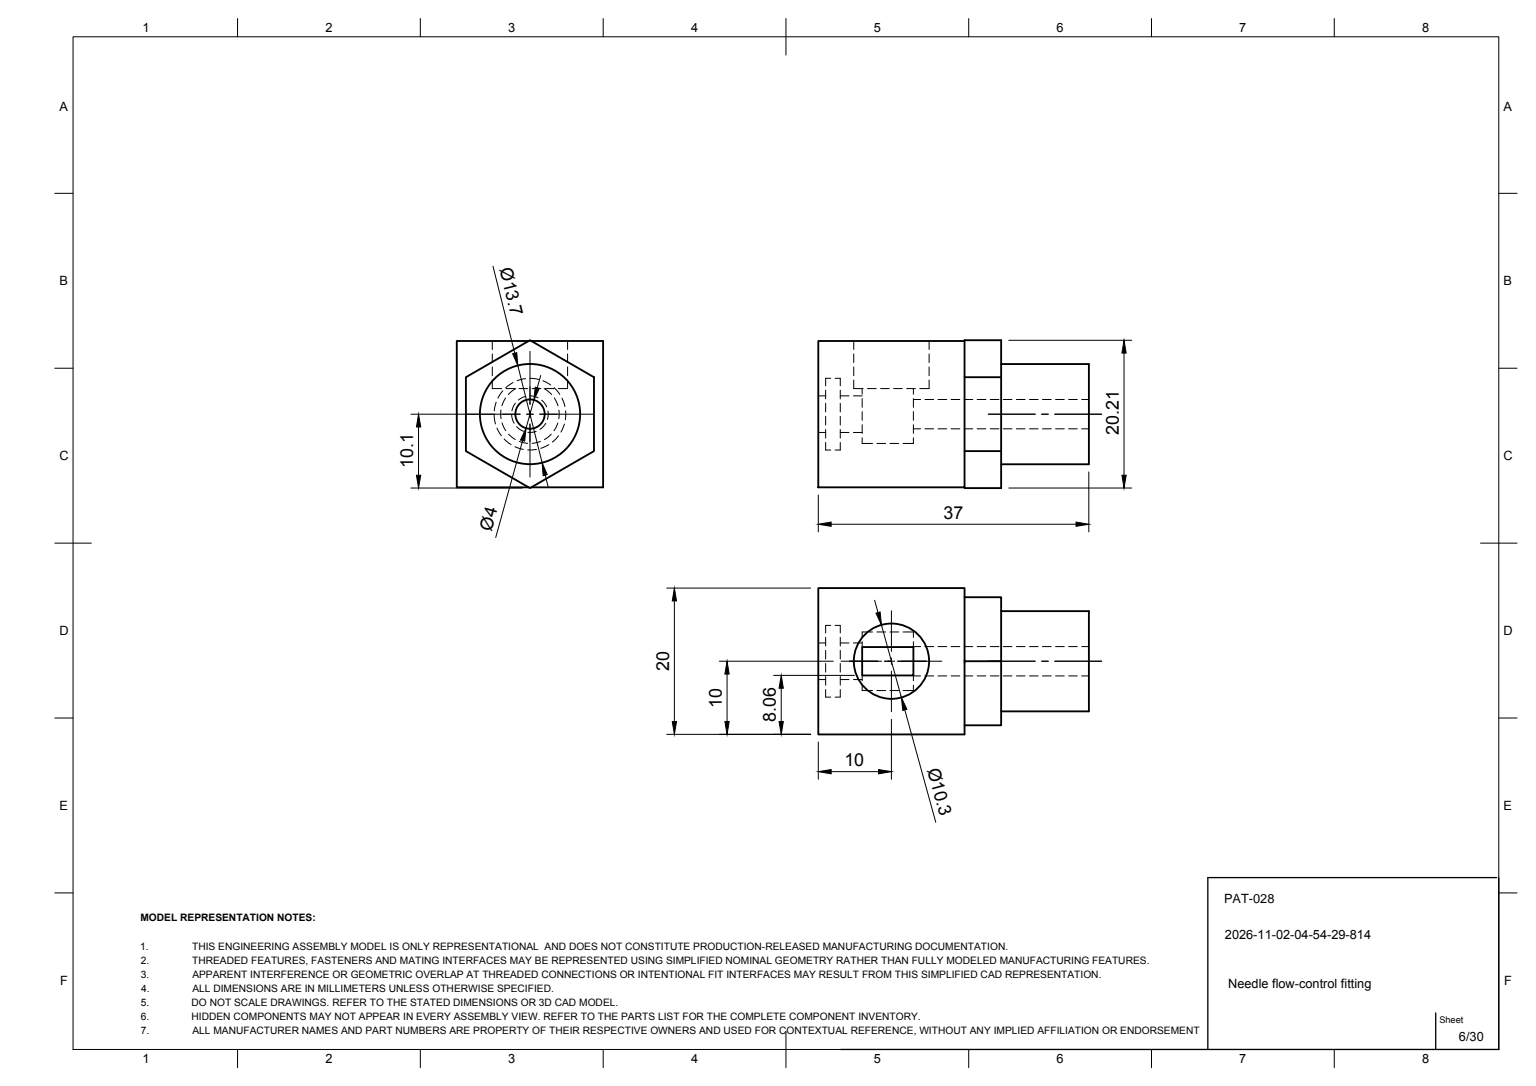
ISO-10303-21;
HEADER;
/* Generated by software containing ST-Developer
 * from STEP Tools, Inc. (www.steptools.com) 
 */

FILE_DESCRIPTION(
/* description */ ('Cylinder foot and clevis mount kit'),
/* implementation_level */ '2;1');

FILE_NAME(
/* name */ 'Needle flow-control fitting.step',
/* time_stamp */ '2026-10-27T20:10:43-07:00',
/* author */ (''),
/* organization */ (''),
/* preprocessor_version */ 'ST-DEVELOPER v20.2',
/* originating_system */ 'Autodesk Translation Framework v15.17.0.0',
/* authorisation */ '');

FILE_SCHEMA (('AUTOMOTIVE_DESIGN { 1 0 10303 214 3 1 1 }'));
ENDSEC;

DATA;
#10=MECHANICAL_DESIGN_GEOMETRIC_PRESENTATION_REPRESENTATION('',(#339),#9102);
#283=SHAPE_REPRESENTATION_RELATIONSHIP('SRR','None',#9230,#311);
#311=ADVANCED_BREP_SHAPE_REPRESENTATION('',(#367),#9073);
#339=STYLED_ITEM('',(#9453),#367);
#367=MANIFOLD_SOLID_BREP('Body1',#4925);
#407=FACE_BOUND('',#1050,.T.);
#408=FACE_BOUND('',#1052,.T.);
#409=FACE_BOUND('',#1056,.T.);
#410=FACE_BOUND('',#1058,.T.);
#411=FACE_BOUND('',#1062,.T.);
#412=FACE_BOUND('',#1066,.T.);
#413=FACE_BOUND('',#1070,.T.);
#414=FACE_BOUND('',#1074,.T.);
#415=FACE_BOUND('',#1085,.T.);
#526=PLANE('',#5339);
#527=PLANE('',#5340);
#528=PLANE('',#5348);
#529=PLANE('',#5350);
#530=PLANE('',#5355);
#531=PLANE('',#5357);
#532=PLANE('',#5358);
#533=PLANE('',#5359);
#534=PLANE('',#5360);
#535=PLANE('',#5361);
#536=PLANE('',#5362);
#537=PLANE('',#5363);
#538=PLANE('',#5364);
#539=PLANE('',#5365);
#540=PLANE('',#5367);
#541=PLANE('',#5368);
#542=PLANE('',#5369);
#543=PLANE('',#5370);
#544=PLANE('',#5371);
#545=PLANE('',#5372);
#546=PLANE('',#5373);
#547=PLANE('',#5378);
#727=FACE_OUTER_BOUND('',#1048,.T.);
#728=FACE_OUTER_BOUND('',#1049,.T.);
#729=FACE_OUTER_BOUND('',#1051,.T.);
#730=FACE_OUTER_BOUND('',#1053,.T.);
#731=FACE_OUTER_BOUND('',#1054,.T.);
#732=FACE_OUTER_BOUND('',#1055,.T.);
#733=FACE_OUTER_BOUND('',#1057,.T.);
#734=FACE_OUTER_BOUND('',#1059,.T.);
#735=FACE_OUTER_BOUND('',#1060,.T.);
#736=FACE_OUTER_BOUND('',#1061,.T.);
#737=FACE_OUTER_BOUND('',#1063,.T.);
#738=FACE_OUTER_BOUND('',#1064,.T.);
#739=FACE_OUTER_BOUND('',#1065,.T.);
#740=FACE_OUTER_BOUND('',#1067,.T.);
#741=FACE_OUTER_BOUND('',#1068,.T.);
#742=FACE_OUTER_BOUND('',#1069,.T.);
#743=FACE_OUTER_BOUND('',#1071,.T.);
#744=FACE_OUTER_BOUND('',#1072,.T.);
#745=FACE_OUTER_BOUND('',#1073,.T.);
#746=FACE_OUTER_BOUND('',#1075,.T.);
#747=FACE_OUTER_BOUND('',#1076,.T.);
#748=FACE_OUTER_BOUND('',#1077,.T.);
#749=FACE_OUTER_BOUND('',#1078,.T.);
#750=FACE_OUTER_BOUND('',#1079,.T.);
#751=FACE_OUTER_BOUND('',#1080,.T.);
#752=FACE_OUTER_BOUND('',#1081,.T.);
#753=FACE_OUTER_BOUND('',#1082,.T.);
#754=FACE_OUTER_BOUND('',#1083,.T.);
#755=FACE_OUTER_BOUND('',#1084,.T.);
#1048=EDGE_LOOP('',(#3449,#3450,#3451,#3452));
#1049=EDGE_LOOP('',(#3453));
#1050=EDGE_LOOP('',(#3454,#3455,#3456,#3457));
#1051=EDGE_LOOP('',(#3458,#3459));
#1052=EDGE_LOOP('',(#3460));
#1053=EDGE_LOOP('',(#3461,#3462,#3463,#3464));
#1054=EDGE_LOOP('',(#3465,#3466,#3467,#3468));
#1055=EDGE_LOOP('',(#3469));
#1056=EDGE_LOOP('',(#3470));
#1057=EDGE_LOOP('',(#3471));
#1058=EDGE_LOOP('',(#3472));
#1059=EDGE_LOOP('',(#3473,#3474,#3475,#3476));
#1060=EDGE_LOOP('',(#3477,#3478,#3479,#3480));
#1061=EDGE_LOOP('',(#3481,#3482));
#1062=EDGE_LOOP('',(#3483));
#1063=EDGE_LOOP('',(#3484,#3485,#3486,#3487,#3488,#3489));
#1064=EDGE_LOOP('',(#3490,#3491,#3492,#3493));
#1065=EDGE_LOOP('',(#3494,#3495,#3496,#3497,#3498,#3499));
#1066=EDGE_LOOP('',(#3500));
#1067=EDGE_LOOP('',(#3501,#3502,#3503,#3504));
#1068=EDGE_LOOP('',(#3505,#3506,#3507,#3508,#3509,#3510));
#1069=EDGE_LOOP('',(#3511,#3512,#3513,#3514));
#1070=EDGE_LOOP('',(#3515));
#1071=EDGE_LOOP('',(#3516,#3517,#3518,#3519,#3520,#3521));
#1072=EDGE_LOOP('',(#3522,#3523,#3524));
#1073=EDGE_LOOP('',(#3525,#3526,#3527,#3528,#3529,#3530));
#1074=EDGE_LOOP('',(#3531));
#1075=EDGE_LOOP('',(#3532,#3533,#3534,#3535));
#1076=EDGE_LOOP('',(#3536,#3537,#3538,#3539,#3540));
#1077=EDGE_LOOP('',(#3541,#3542,#3543,#3544,#3545));
#1078=EDGE_LOOP('',(#3546,#3547,#3548,#3549));
#1079=EDGE_LOOP('',(#3550,#3551,#3552,#3553,#3554));
#1080=EDGE_LOOP('',(#3555,#3556,#3557,#3558,#3559));
#1081=EDGE_LOOP('',(#3560,#3561,#3562));
#1082=EDGE_LOOP('',(#3563,#3564,#3565,#3566));
#1083=EDGE_LOOP('',(#3567,#3568,#3569,#3570));
#1084=EDGE_LOOP('',(#3571));
#1085=EDGE_LOOP('',(#3572));
#1440=LINE('',#7643,#1789);
#1441=LINE('',#7648,#1790);
#1442=LINE('',#7650,#1791);
#1443=LINE('',#7652,#1792);
#1444=LINE('',#7653,#1793);
#1445=LINE('',#7664,#1794);
#1446=LINE('',#7673,#1795);
#1447=LINE('',#7676,#1796);
#1448=LINE('',#7684,#1797);
#1449=LINE('',#7686,#1798);
#1450=LINE('',#7688,#1799);
#1451=LINE('',#7690,#1800);
#1452=LINE('',#7692,#1801);
#1453=LINE('',#7693,#1802);
#1454=LINE('',#7697,#1803);
#1455=LINE('',#7699,#1804);
#1456=LINE('',#7701,#1805);
#1457=LINE('',#7702,#1806);
#1458=LINE('',#7705,#1807);
#1459=LINE('',#7706,#1808);
#1460=LINE('',#7708,#1809);
#1461=LINE('',#7709,#1810);
#1462=LINE('',#7712,#1811);
#1463=LINE('',#7713,#1812);
#1464=LINE('',#7716,#1813);
#1465=LINE('',#7717,#1814);
#1466=LINE('',#7718,#1815);
#1467=LINE('',#7722,#1816);
#1468=LINE('',#7724,#1817);
#1469=LINE('',#7725,#1818);
#1470=LINE('',#7728,#1819);
#1471=LINE('',#7729,#1820);
#1472=LINE('',#7733,#1821);
#1473=LINE('',#7735,#1822);
#1474=LINE('',#7737,#1823);
#1475=LINE('',#7739,#1824);
#1476=LINE('',#7741,#1825);
#1477=LINE('',#7742,#1826);
#1478=LINE('',#7746,#1827);
#1479=LINE('',#7747,#1828);
#1480=LINE('',#7750,#1829);
#1481=LINE('',#7751,#1830);
#1482=LINE('',#7753,#1831);
#1483=LINE('',#7754,#1832);
#1484=LINE('',#7756,#1833);
#1485=LINE('',#7758,#1834);
#1486=LINE('',#7763,#1835);
#1487=LINE('',#7767,#1836);
#1789=VECTOR('',#6071,0.515);
#1790=VECTOR('',#6076,1.);
#1791=VECTOR('',#6077,1.);
#1792=VECTOR('',#6078,1.);
#1793=VECTOR('',#6079,1.);
#1794=VECTOR('',#6094,0.49);
#1795=VECTOR('',#6107,0.25);
#1796=VECTOR('',#6110,0.25);
#1797=VECTOR('',#6119,1.);
#1798=VECTOR('',#6120,1.);
#1799=VECTOR('',#6121,1.);
#1800=VECTOR('',#6122,1.);
#1801=VECTOR('',#6123,1.);
#1802=VECTOR('',#6124,1.);
#1803=VECTOR('',#6127,1.);
#1804=VECTOR('',#6128,1.);
#1805=VECTOR('',#6129,1.);
#1806=VECTOR('',#6130,1.);
#1807=VECTOR('',#6133,1.);
#1808=VECTOR('',#6134,1.);
#1809=VECTOR('',#6135,1.);
#1810=VECTOR('',#6136,1.);
#1811=VECTOR('',#6139,1.);
#1812=VECTOR('',#6140,1.);
#1813=VECTOR('',#6143,1.);
#1814=VECTOR('',#6144,1.);
#1815=VECTOR('',#6145,1.);
#1816=VECTOR('',#6150,1.);
#1817=VECTOR('',#6151,1.);
#1818=VECTOR('',#6152,1.);
#1819=VECTOR('',#6155,1.);
#1820=VECTOR('',#6156,1.);
#1821=VECTOR('',#6159,1.);
#1822=VECTOR('',#6160,1.);
#1823=VECTOR('',#6161,1.);
#1824=VECTOR('',#6162,1.);
#1825=VECTOR('',#6163,1.);
#1826=VECTOR('',#6164,1.);
#1827=VECTOR('',#6169,1.);
#1828=VECTOR('',#6170,1.);
#1829=VECTOR('',#6173,1.);
#1830=VECTOR('',#6174,1.);
#1831=VECTOR('',#6177,1.);
#1832=VECTOR('',#6178,1.);
#1833=VECTOR('',#6181,1.);
#1834=VECTOR('',#6184,1.);
#1835=VECTOR('',#6191,0.2);
#1836=VECTOR('',#6196,0.685);
#2138=CIRCLE('',#5337,0.515);
#2139=CIRCLE('',#5338,0.515);
#2140=CIRCLE('',#5341,0.4);
#2141=CIRCLE('',#5342,0.25);
#2142=CIRCLE('',#5344,0.4);
#2143=CIRCLE('',#5346,0.49);
#2144=CIRCLE('',#5347,0.49);
#2145=CIRCLE('',#5349,0.25);
#2146=CIRCLE('',#5351,0.25);
#2147=CIRCLE('',#5354,0.25);
#2148=CIRCLE('',#5356,0.2);
#2149=CIRCLE('',#5366,0.685);
#2150=CIRCLE('',#5375,0.2);
#2151=CIRCLE('',#5377,0.685);
#2368=VERTEX_POINT('',#7640);
#2369=VERTEX_POINT('',#7642);
#2370=VERTEX_POINT('',#7646);
#2371=VERTEX_POINT('',#7647);
#2372=VERTEX_POINT('',#7649);
#2373=VERTEX_POINT('',#7651);
#2374=VERTEX_POINT('',#7656);
#2375=VERTEX_POINT('',#7661);
#2376=VERTEX_POINT('',#7663);
#2377=VERTEX_POINT('',#7667);
#2378=VERTEX_POINT('',#7670);
#2379=VERTEX_POINT('',#7675);
#2380=VERTEX_POINT('',#7679);
#2381=VERTEX_POINT('',#7682);
#2382=VERTEX_POINT('',#7683);
#2383=VERTEX_POINT('',#7685);
#2384=VERTEX_POINT('',#7687);
#2385=VERTEX_POINT('',#7689);
#2386=VERTEX_POINT('',#7691);
#2387=VERTEX_POINT('',#7695);
#2388=VERTEX_POINT('',#7696);
#2389=VERTEX_POINT('',#7698);
#2390=VERTEX_POINT('',#7700);
#2391=VERTEX_POINT('',#7704);
#2392=VERTEX_POINT('',#7707);
#2393=VERTEX_POINT('',#7711);
#2394=VERTEX_POINT('',#7715);
#2395=VERTEX_POINT('',#7721);
#2396=VERTEX_POINT('',#7723);
#2397=VERTEX_POINT('',#7727);
#2398=VERTEX_POINT('',#7731);
#2399=VERTEX_POINT('',#7732);
#2400=VERTEX_POINT('',#7734);
#2401=VERTEX_POINT('',#7736);
#2402=VERTEX_POINT('',#7738);
#2403=VERTEX_POINT('',#7740);
#2404=VERTEX_POINT('',#7743);
#2405=VERTEX_POINT('',#7749);
#2406=VERTEX_POINT('',#7762);
#2407=VERTEX_POINT('',#7766);
#2779=EDGE_CURVE('',#2368,#2368,#2138,.T.);
#2780=EDGE_CURVE('',#2368,#2369,#1440,.T.);
#2781=EDGE_CURVE('',#2369,#2369,#2139,.T.);
#2782=EDGE_CURVE('',#2370,#2371,#1441,.T.);
#2783=EDGE_CURVE('',#2372,#2370,#1442,.T.);
#2784=EDGE_CURVE('',#2373,#2372,#1443,.T.);
#2785=EDGE_CURVE('',#2371,#2373,#1444,.T.);
#2786=EDGE_CURVE('',#2372,#2370,#2140,.T.);
#2787=EDGE_CURVE('',#2374,#2374,#2141,.T.);
#2788=EDGE_CURVE('',#2373,#2371,#2142,.T.);
#2789=EDGE_CURVE('',#2375,#2375,#2143,.T.);
#2790=EDGE_CURVE('',#2375,#2376,#1445,.T.);
#2791=EDGE_CURVE('',#2376,#2376,#2144,.T.);
#2792=EDGE_CURVE('',#2377,#2377,#2145,.T.);
#2793=EDGE_CURVE('',#2378,#2378,#2146,.T.);
#2794=EDGE_CURVE('',#2374,#2378,#1446,.T.);
#2795=EDGE_CURVE('',#2377,#2379,#1447,.T.);
#2796=EDGE_CURVE('',#2379,#2379,#2147,.T.);
#2797=EDGE_CURVE('',#2380,#2380,#2148,.T.);
#2798=EDGE_CURVE('',#2381,#2382,#1448,.T.);
#2799=EDGE_CURVE('',#2382,#2383,#1449,.T.);
#2800=EDGE_CURVE('',#2383,#2384,#1450,.T.);
#2801=EDGE_CURVE('',#2385,#2384,#1451,.T.);
#2802=EDGE_CURVE('',#2386,#2385,#1452,.T.);
#2803=EDGE_CURVE('',#2381,#2386,#1453,.T.);
#2804=EDGE_CURVE('',#2387,#2388,#1454,.T.);
#2805=EDGE_CURVE('',#2388,#2389,#1455,.T.);
#2806=EDGE_CURVE('',#2390,#2389,#1456,.T.);
#2807=EDGE_CURVE('',#2387,#2390,#1457,.T.);
#2808=EDGE_CURVE('',#2391,#2384,#1458,.T.);
#2809=EDGE_CURVE('',#2391,#2387,#1459,.T.);
#2810=EDGE_CURVE('',#2392,#2390,#1460,.T.);
#2811=EDGE_CURVE('',#2385,#2392,#1461,.T.);
#2812=EDGE_CURVE('',#2393,#2392,#1462,.T.);
#2813=EDGE_CURVE('',#2386,#2393,#1463,.T.);
#2814=EDGE_CURVE('',#2388,#2394,#1464,.T.);
#2815=EDGE_CURVE('',#2381,#2394,#1465,.T.);
#2816=EDGE_CURVE('',#2389,#2393,#1466,.T.);
#2817=EDGE_CURVE('',#2395,#2394,#1467,.T.);
#2818=EDGE_CURVE('',#2391,#2396,#1468,.T.);
#2819=EDGE_CURVE('',#2396,#2395,#1469,.T.);
#2820=EDGE_CURVE('',#2384,#2397,#1470,.T.);
#2821=EDGE_CURVE('',#2397,#2391,#1471,.T.);
#2822=EDGE_CURVE('',#2398,#2399,#1472,.T.);
#2823=EDGE_CURVE('',#2400,#2398,#1473,.T.);
#2824=EDGE_CURVE('',#2401,#2400,#1474,.T.);
#2825=EDGE_CURVE('',#2402,#2401,#1475,.T.);
#2826=EDGE_CURVE('',#2403,#2402,#1476,.T.);
#2827=EDGE_CURVE('',#2399,#2403,#1477,.T.);
#2828=EDGE_CURVE('',#2404,#2404,#2149,.T.);
#2829=EDGE_CURVE('',#2398,#2383,#1478,.T.);
#2830=EDGE_CURVE('',#2400,#2382,#1479,.T.);
#2831=EDGE_CURVE('',#2405,#2381,#1480,.T.);
#2832=EDGE_CURVE('',#2401,#2405,#1481,.T.);
#2833=EDGE_CURVE('',#2394,#2405,#1482,.T.);
#2834=EDGE_CURVE('',#2402,#2395,#1483,.T.);
#2835=EDGE_CURVE('',#2403,#2396,#1484,.T.);
#2836=EDGE_CURVE('',#2399,#2397,#1485,.T.);
#2837=EDGE_CURVE('',#2380,#2406,#1486,.T.);
#2838=EDGE_CURVE('',#2406,#2406,#2150,.T.);
#2839=EDGE_CURVE('',#2404,#2407,#1487,.T.);
#2840=EDGE_CURVE('',#2407,#2407,#2151,.T.);
#3449=ORIENTED_EDGE('',*,*,#2779,.F.);
#3450=ORIENTED_EDGE('',*,*,#2780,.T.);
#3451=ORIENTED_EDGE('',*,*,#2781,.F.);
#3452=ORIENTED_EDGE('',*,*,#2780,.F.);
#3453=ORIENTED_EDGE('',*,*,#2779,.T.);
#3454=ORIENTED_EDGE('',*,*,#2782,.F.);
#3455=ORIENTED_EDGE('',*,*,#2783,.F.);
#3456=ORIENTED_EDGE('',*,*,#2784,.F.);
#3457=ORIENTED_EDGE('',*,*,#2785,.F.);
#3458=ORIENTED_EDGE('',*,*,#2783,.T.);
#3459=ORIENTED_EDGE('',*,*,#2786,.F.);
#3460=ORIENTED_EDGE('',*,*,#2787,.T.);
#3461=ORIENTED_EDGE('',*,*,#2784,.T.);
#3462=ORIENTED_EDGE('',*,*,#2786,.T.);
#3463=ORIENTED_EDGE('',*,*,#2782,.T.);
#3464=ORIENTED_EDGE('',*,*,#2788,.F.);
#3465=ORIENTED_EDGE('',*,*,#2789,.F.);
#3466=ORIENTED_EDGE('',*,*,#2790,.T.);
#3467=ORIENTED_EDGE('',*,*,#2791,.T.);
#3468=ORIENTED_EDGE('',*,*,#2790,.F.);
#3469=ORIENTED_EDGE('',*,*,#2791,.F.);
#3470=ORIENTED_EDGE('',*,*,#2792,.F.);
#3471=ORIENTED_EDGE('',*,*,#2789,.T.);
#3472=ORIENTED_EDGE('',*,*,#2793,.F.);
#3473=ORIENTED_EDGE('',*,*,#2787,.F.);
#3474=ORIENTED_EDGE('',*,*,#2794,.T.);
#3475=ORIENTED_EDGE('',*,*,#2793,.T.);
#3476=ORIENTED_EDGE('',*,*,#2794,.F.);
#3477=ORIENTED_EDGE('',*,*,#2792,.T.);
#3478=ORIENTED_EDGE('',*,*,#2795,.T.);
#3479=ORIENTED_EDGE('',*,*,#2796,.F.);
#3480=ORIENTED_EDGE('',*,*,#2795,.F.);
#3481=ORIENTED_EDGE('',*,*,#2785,.T.);
#3482=ORIENTED_EDGE('',*,*,#2788,.T.);
#3483=ORIENTED_EDGE('',*,*,#2797,.F.);
#3484=ORIENTED_EDGE('',*,*,#2798,.T.);
#3485=ORIENTED_EDGE('',*,*,#2799,.T.);
#3486=ORIENTED_EDGE('',*,*,#2800,.T.);
#3487=ORIENTED_EDGE('',*,*,#2801,.F.);
#3488=ORIENTED_EDGE('',*,*,#2802,.F.);
#3489=ORIENTED_EDGE('',*,*,#2803,.F.);
#3490=ORIENTED_EDGE('',*,*,#2804,.T.);
#3491=ORIENTED_EDGE('',*,*,#2805,.T.);
#3492=ORIENTED_EDGE('',*,*,#2806,.F.);
#3493=ORIENTED_EDGE('',*,*,#2807,.F.);
#3494=ORIENTED_EDGE('',*,*,#2801,.T.);
#3495=ORIENTED_EDGE('',*,*,#2808,.F.);
#3496=ORIENTED_EDGE('',*,*,#2809,.T.);
#3497=ORIENTED_EDGE('',*,*,#2807,.T.);
#3498=ORIENTED_EDGE('',*,*,#2810,.F.);
#3499=ORIENTED_EDGE('',*,*,#2811,.F.);
#3500=ORIENTED_EDGE('',*,*,#2781,.T.);
#3501=ORIENTED_EDGE('',*,*,#2802,.T.);
#3502=ORIENTED_EDGE('',*,*,#2811,.T.);
#3503=ORIENTED_EDGE('',*,*,#2812,.F.);
#3504=ORIENTED_EDGE('',*,*,#2813,.F.);
#3505=ORIENTED_EDGE('',*,*,#2814,.T.);
#3506=ORIENTED_EDGE('',*,*,#2815,.F.);
#3507=ORIENTED_EDGE('',*,*,#2803,.T.);
#3508=ORIENTED_EDGE('',*,*,#2813,.T.);
#3509=ORIENTED_EDGE('',*,*,#2816,.F.);
#3510=ORIENTED_EDGE('',*,*,#2805,.F.);
#3511=ORIENTED_EDGE('',*,*,#2816,.T.);
#3512=ORIENTED_EDGE('',*,*,#2812,.T.);
#3513=ORIENTED_EDGE('',*,*,#2810,.T.);
#3514=ORIENTED_EDGE('',*,*,#2806,.T.);
#3515=ORIENTED_EDGE('',*,*,#2796,.T.);
#3516=ORIENTED_EDGE('',*,*,#2817,.T.);
#3517=ORIENTED_EDGE('',*,*,#2814,.F.);
#3518=ORIENTED_EDGE('',*,*,#2804,.F.);
#3519=ORIENTED_EDGE('',*,*,#2809,.F.);
#3520=ORIENTED_EDGE('',*,*,#2818,.T.);
#3521=ORIENTED_EDGE('',*,*,#2819,.T.);
#3522=ORIENTED_EDGE('',*,*,#2808,.T.);
#3523=ORIENTED_EDGE('',*,*,#2820,.T.);
#3524=ORIENTED_EDGE('',*,*,#2821,.T.);
#3525=ORIENTED_EDGE('',*,*,#2822,.F.);
#3526=ORIENTED_EDGE('',*,*,#2823,.F.);
#3527=ORIENTED_EDGE('',*,*,#2824,.F.);
#3528=ORIENTED_EDGE('',*,*,#2825,.F.);
#3529=ORIENTED_EDGE('',*,*,#2826,.F.);
#3530=ORIENTED_EDGE('',*,*,#2827,.F.);
#3531=ORIENTED_EDGE('',*,*,#2828,.T.);
#3532=ORIENTED_EDGE('',*,*,#2823,.T.);
#3533=ORIENTED_EDGE('',*,*,#2829,.T.);
#3534=ORIENTED_EDGE('',*,*,#2799,.F.);
#3535=ORIENTED_EDGE('',*,*,#2830,.F.);
#3536=ORIENTED_EDGE('',*,*,#2824,.T.);
#3537=ORIENTED_EDGE('',*,*,#2830,.T.);
#3538=ORIENTED_EDGE('',*,*,#2798,.F.);
#3539=ORIENTED_EDGE('',*,*,#2831,.F.);
#3540=ORIENTED_EDGE('',*,*,#2832,.F.);
#3541=ORIENTED_EDGE('',*,*,#2825,.T.);
#3542=ORIENTED_EDGE('',*,*,#2832,.T.);
#3543=ORIENTED_EDGE('',*,*,#2833,.F.);
#3544=ORIENTED_EDGE('',*,*,#2817,.F.);
#3545=ORIENTED_EDGE('',*,*,#2834,.F.);
#3546=ORIENTED_EDGE('',*,*,#2826,.T.);
#3547=ORIENTED_EDGE('',*,*,#2834,.T.);
#3548=ORIENTED_EDGE('',*,*,#2819,.F.);
#3549=ORIENTED_EDGE('',*,*,#2835,.F.);
#3550=ORIENTED_EDGE('',*,*,#2827,.T.);
#3551=ORIENTED_EDGE('',*,*,#2835,.T.);
#3552=ORIENTED_EDGE('',*,*,#2818,.F.);
#3553=ORIENTED_EDGE('',*,*,#2821,.F.);
#3554=ORIENTED_EDGE('',*,*,#2836,.F.);
#3555=ORIENTED_EDGE('',*,*,#2822,.T.);
#3556=ORIENTED_EDGE('',*,*,#2836,.T.);
#3557=ORIENTED_EDGE('',*,*,#2820,.F.);
#3558=ORIENTED_EDGE('',*,*,#2800,.F.);
#3559=ORIENTED_EDGE('',*,*,#2829,.F.);
#3560=ORIENTED_EDGE('',*,*,#2815,.T.);
#3561=ORIENTED_EDGE('',*,*,#2833,.T.);
#3562=ORIENTED_EDGE('',*,*,#2831,.T.);
#3563=ORIENTED_EDGE('',*,*,#2797,.T.);
#3564=ORIENTED_EDGE('',*,*,#2837,.T.);
#3565=ORIENTED_EDGE('',*,*,#2838,.T.);
#3566=ORIENTED_EDGE('',*,*,#2837,.F.);
#3567=ORIENTED_EDGE('',*,*,#2828,.F.);
#3568=ORIENTED_EDGE('',*,*,#2839,.T.);
#3569=ORIENTED_EDGE('',*,*,#2840,.T.);
#3570=ORIENTED_EDGE('',*,*,#2839,.F.);
#3571=ORIENTED_EDGE('',*,*,#2840,.F.);
#3572=ORIENTED_EDGE('',*,*,#2838,.F.);
#4536=CYLINDRICAL_SURFACE('',#5336,0.515);
#4537=CYLINDRICAL_SURFACE('',#5343,0.4);
#4538=CYLINDRICAL_SURFACE('',#5345,0.49);
#4539=CYLINDRICAL_SURFACE('',#5352,0.25);
#4540=CYLINDRICAL_SURFACE('',#5353,0.25);
#4541=CYLINDRICAL_SURFACE('',#5374,0.2);
#4542=CYLINDRICAL_SURFACE('',#5376,0.685);
#4650=ADVANCED_FACE('',(#727),#4536,.F.);
#4651=ADVANCED_FACE('',(#728,#407),#526,.T.);
#4652=ADVANCED_FACE('',(#729,#408),#527,.F.);
#4653=ADVANCED_FACE('',(#730),#4537,.F.);
#4654=ADVANCED_FACE('',(#731),#4538,.F.);
#4655=ADVANCED_FACE('',(#732,#409),#528,.F.);
#4656=ADVANCED_FACE('',(#733,#410),#529,.T.);
#4657=ADVANCED_FACE('',(#734),#4539,.F.);
#4658=ADVANCED_FACE('',(#735),#4540,.F.);
#4659=ADVANCED_FACE('',(#736,#411),#530,.T.);
#4660=ADVANCED_FACE('',(#737),#531,.F.);
#4661=ADVANCED_FACE('',(#738),#532,.T.);
#4662=ADVANCED_FACE('',(#739,#412),#533,.T.);
#4663=ADVANCED_FACE('',(#740),#534,.T.);
#4664=ADVANCED_FACE('',(#741),#535,.T.);
#4665=ADVANCED_FACE('',(#742,#413),#536,.T.);
#4666=ADVANCED_FACE('',(#743),#537,.F.);
#4667=ADVANCED_FACE('',(#744),#538,.T.);
#4668=ADVANCED_FACE('',(#745,#414),#539,.F.);
#4669=ADVANCED_FACE('',(#746),#540,.T.);
#4670=ADVANCED_FACE('',(#747),#541,.T.);
#4671=ADVANCED_FACE('',(#748),#542,.T.);
#4672=ADVANCED_FACE('',(#749),#543,.T.);
#4673=ADVANCED_FACE('',(#750),#544,.T.);
#4674=ADVANCED_FACE('',(#751),#545,.T.);
#4675=ADVANCED_FACE('',(#752),#546,.T.);
#4676=ADVANCED_FACE('',(#753),#4541,.F.);
#4677=ADVANCED_FACE('',(#754),#4542,.T.);
#4678=ADVANCED_FACE('',(#755,#415),#547,.F.);
#4925=CLOSED_SHELL('',(#4650,#4651,#4652,#4653,#4654,#4655,#4656,#4657,
#4658,#4659,#4660,#4661,#4662,#4663,#4664,#4665,#4666,#4667,#4668,#4669,
#4670,#4671,#4672,#4673,#4674,#4675,#4676,#4677,#4678));
#5335=AXIS2_PLACEMENT_3D('',#7638,#6065,#6066);
#5336=AXIS2_PLACEMENT_3D('',#7639,#6067,#6068);
#5337=AXIS2_PLACEMENT_3D('',#7641,#6069,#6070);
#5338=AXIS2_PLACEMENT_3D('',#7644,#6072,#6073);
#5339=AXIS2_PLACEMENT_3D('',#7645,#6074,#6075);
#5340=AXIS2_PLACEMENT_3D('',#7654,#6080,#6081);
#5341=AXIS2_PLACEMENT_3D('',#7655,#6082,#6083);
#5342=AXIS2_PLACEMENT_3D('',#7657,#6084,#6085);
#5343=AXIS2_PLACEMENT_3D('',#7658,#6086,#6087);
#5344=AXIS2_PLACEMENT_3D('',#7659,#6088,#6089);
#5345=AXIS2_PLACEMENT_3D('',#7660,#6090,#6091);
#5346=AXIS2_PLACEMENT_3D('',#7662,#6092,#6093);
#5347=AXIS2_PLACEMENT_3D('',#7665,#6095,#6096);
#5348=AXIS2_PLACEMENT_3D('',#7666,#6097,#6098);
#5349=AXIS2_PLACEMENT_3D('',#7668,#6099,#6100);
#5350=AXIS2_PLACEMENT_3D('',#7669,#6101,#6102);
#5351=AXIS2_PLACEMENT_3D('',#7671,#6103,#6104);
#5352=AXIS2_PLACEMENT_3D('',#7672,#6105,#6106);
#5353=AXIS2_PLACEMENT_3D('',#7674,#6108,#6109);
#5354=AXIS2_PLACEMENT_3D('',#7677,#6111,#6112);
#5355=AXIS2_PLACEMENT_3D('',#7678,#6113,#6114);
#5356=AXIS2_PLACEMENT_3D('',#7680,#6115,#6116);
#5357=AXIS2_PLACEMENT_3D('',#7681,#6117,#6118);
#5358=AXIS2_PLACEMENT_3D('',#7694,#6125,#6126);
#5359=AXIS2_PLACEMENT_3D('',#7703,#6131,#6132);
#5360=AXIS2_PLACEMENT_3D('',#7710,#6137,#6138);
#5361=AXIS2_PLACEMENT_3D('',#7714,#6141,#6142);
#5362=AXIS2_PLACEMENT_3D('',#7719,#6146,#6147);
#5363=AXIS2_PLACEMENT_3D('',#7720,#6148,#6149);
#5364=AXIS2_PLACEMENT_3D('',#7726,#6153,#6154);
#5365=AXIS2_PLACEMENT_3D('',#7730,#6157,#6158);
#5366=AXIS2_PLACEMENT_3D('',#7744,#6165,#6166);
#5367=AXIS2_PLACEMENT_3D('',#7745,#6167,#6168);
#5368=AXIS2_PLACEMENT_3D('',#7748,#6171,#6172);
#5369=AXIS2_PLACEMENT_3D('',#7752,#6175,#6176);
#5370=AXIS2_PLACEMENT_3D('',#7755,#6179,#6180);
#5371=AXIS2_PLACEMENT_3D('',#7757,#6182,#6183);
#5372=AXIS2_PLACEMENT_3D('',#7759,#6185,#6186);
#5373=AXIS2_PLACEMENT_3D('',#7760,#6187,#6188);
#5374=AXIS2_PLACEMENT_3D('',#7761,#6189,#6190);
#5375=AXIS2_PLACEMENT_3D('',#7764,#6192,#6193);
#5376=AXIS2_PLACEMENT_3D('',#7765,#6194,#6195);
#5377=AXIS2_PLACEMENT_3D('',#7768,#6197,#6198);
#5378=AXIS2_PLACEMENT_3D('',#7769,#6199,#6200);
#6065=DIRECTION('axis',(0.,0.,1.));
#6066=DIRECTION('refdir',(1.,0.,0.));
#6067=DIRECTION('center_axis',(1.,0.,0.));
#6068=DIRECTION('ref_axis',(0.,0.,-1.));
#6069=DIRECTION('center_axis',(1.,0.,0.));
#6070=DIRECTION('ref_axis',(0.,0.,-1.));
#6071=DIRECTION('',(1.,0.,0.));
#6072=DIRECTION('center_axis',(-1.,0.,0.));
#6073=DIRECTION('ref_axis',(0.,0.,-1.));
#6074=DIRECTION('center_axis',(1.,0.,0.));
#6075=DIRECTION('ref_axis',(0.,0.,-1.));
#6076=DIRECTION('',(0.,0.,-1.));
#6077=DIRECTION('',(0.,-1.,0.));
#6078=DIRECTION('',(0.,0.,1.));
#6079=DIRECTION('',(0.,1.,0.));
#6080=DIRECTION('center_axis',(0.,0.,1.));
#6081=DIRECTION('ref_axis',(1.,0.,0.));
#6082=DIRECTION('center_axis',(0.,0.,1.));
#6083=DIRECTION('ref_axis',(1.,0.,0.));
#6084=DIRECTION('center_axis',(0.,0.,1.));
#6085=DIRECTION('ref_axis',(1.,0.,0.));
#6086=DIRECTION('center_axis',(0.,0.,1.));
#6087=DIRECTION('ref_axis',(-1.,1.22464679914735E-16,0.));
#6088=DIRECTION('center_axis',(0.,0.,1.));
#6089=DIRECTION('ref_axis',(1.,0.,0.));
#6090=DIRECTION('center_axis',(0.,0.,1.));
#6091=DIRECTION('ref_axis',(1.,0.,0.));
#6092=DIRECTION('center_axis',(0.,0.,1.));
#6093=DIRECTION('ref_axis',(1.,0.,0.));
#6094=DIRECTION('',(0.,0.,1.));
#6095=DIRECTION('center_axis',(0.,0.,1.));
#6096=DIRECTION('ref_axis',(1.,0.,0.));
#6097=DIRECTION('center_axis',(0.,0.,1.));
#6098=DIRECTION('ref_axis',(1.,0.,0.));
#6099=DIRECTION('center_axis',(0.,0.,-1.));
#6100=DIRECTION('ref_axis',(1.,0.,0.));
#6101=DIRECTION('center_axis',(0.,0.,1.));
#6102=DIRECTION('ref_axis',(1.,0.,0.));
#6103=DIRECTION('center_axis',(0.,0.,1.));
#6104=DIRECTION('ref_axis',(1.,0.,0.));
#6105=DIRECTION('center_axis',(0.,0.,1.));
#6106=DIRECTION('ref_axis',(1.,0.,0.));
#6107=DIRECTION('',(0.,0.,1.));
#6108=DIRECTION('center_axis',(0.,0.,1.));
#6109=DIRECTION('ref_axis',(1.,0.,0.));
#6110=DIRECTION('',(0.,0.,1.));
#6111=DIRECTION('center_axis',(0.,0.,-1.));
#6112=DIRECTION('ref_axis',(1.,0.,0.));
#6113=DIRECTION('center_axis',(0.,0.,1.));
#6114=DIRECTION('ref_axis',(1.,0.,0.));
#6115=DIRECTION('center_axis',(0.,0.,1.));
#6116=DIRECTION('ref_axis',(1.,0.,0.));
#6117=DIRECTION('center_axis',(0.,0.,1.));
#6118=DIRECTION('ref_axis',(1.,0.,0.));
#6119=DIRECTION('',(0.5,-0.866025403784439,0.));
#6120=DIRECTION('',(1.,-3.43386193997065E-16,0.));
#6121=DIRECTION('',(0.5,0.866025403784439,0.));
#6122=DIRECTION('',(0.,1.,0.));
#6123=DIRECTION('',(1.,0.,0.));
#6124=DIRECTION('',(0.,-1.,0.));
#6125=DIRECTION('center_axis',(0.,1.,0.));
#6126=DIRECTION('ref_axis',(-1.,0.,0.));
#6127=DIRECTION('',(-1.,0.,0.));
#6128=DIRECTION('',(0.,0.,1.));
#6129=DIRECTION('',(-1.,0.,0.));
#6130=DIRECTION('',(0.,0.,1.));
#6131=DIRECTION('center_axis',(1.,0.,0.));
#6132=DIRECTION('ref_axis',(0.,1.,0.));
#6133=DIRECTION('',(0.,-1.,0.));
#6134=DIRECTION('',(0.,1.,0.));
#6135=DIRECTION('',(0.,1.,0.));
#6136=DIRECTION('',(0.,0.,1.));
#6137=DIRECTION('center_axis',(0.,-1.,0.));
#6138=DIRECTION('ref_axis',(1.,0.,0.));
#6139=DIRECTION('',(1.,0.,0.));
#6140=DIRECTION('',(0.,0.,1.));
#6141=DIRECTION('center_axis',(-1.,0.,0.));
#6142=DIRECTION('ref_axis',(0.,-1.,0.));
#6143=DIRECTION('',(0.,-1.,0.));
#6144=DIRECTION('',(0.,1.,0.));
#6145=DIRECTION('',(0.,-1.,0.));
#6146=DIRECTION('center_axis',(0.,0.,1.));
#6147=DIRECTION('ref_axis',(1.,0.,0.));
#6148=DIRECTION('center_axis',(0.,0.,1.));
#6149=DIRECTION('ref_axis',(1.,0.,0.));
#6150=DIRECTION('',(-0.5,-0.866025403784439,0.));
#6151=DIRECTION('',(-0.5,0.866025403784439,0.));
#6152=DIRECTION('',(-1.,0.,0.));
#6153=DIRECTION('center_axis',(0.,0.,1.));
#6154=DIRECTION('ref_axis',(1.,0.,0.));
#6155=DIRECTION('',(0.5,0.866025403784439,0.));
#6156=DIRECTION('',(-0.5,0.866025403784439,0.));
#6157=DIRECTION('center_axis',(0.,0.,1.));
#6158=DIRECTION('ref_axis',(1.,0.,0.));
#6159=DIRECTION('',(0.5,0.866025403784439,0.));
#6160=DIRECTION('',(1.,-3.43386193997065E-16,0.));
#6161=DIRECTION('',(0.5,-0.866025403784439,0.));
#6162=DIRECTION('',(-0.5,-0.866025403784438,0.));
#6163=DIRECTION('',(-1.,0.,0.));
#6164=DIRECTION('',(-0.5,0.866025403784439,0.));
#6165=DIRECTION('center_axis',(0.,0.,1.));
#6166=DIRECTION('ref_axis',(1.,0.,0.));
#6167=DIRECTION('center_axis',(-3.43386193997065E-16,-1.,0.));
#6168=DIRECTION('ref_axis',(1.,-3.43386193997065E-16,0.));
#6169=DIRECTION('',(0.,0.,1.));
#6170=DIRECTION('',(0.,0.,1.));
#6171=DIRECTION('center_axis',(-0.866025403784439,-0.5,0.));
#6172=DIRECTION('ref_axis',(0.5,-0.866025403784439,0.));
#6173=DIRECTION('',(0.5,-0.866025403784439,0.));
#6174=DIRECTION('',(0.,0.,1.));
#6175=DIRECTION('center_axis',(-0.866025403784439,0.5,0.));
#6176=DIRECTION('ref_axis',(-0.5,-0.866025403784439,0.));
#6177=DIRECTION('',(-0.5,-0.866025403784438,0.));
#6178=DIRECTION('',(0.,0.,1.));
#6179=DIRECTION('center_axis',(0.,1.,0.));
#6180=DIRECTION('ref_axis',(-1.,0.,0.));
#6181=DIRECTION('',(0.,0.,1.));
#6182=DIRECTION('center_axis',(0.866025403784439,0.5,0.));
#6183=DIRECTION('ref_axis',(-0.5,0.866025403784439,0.));
#6184=DIRECTION('',(0.,0.,1.));
#6185=DIRECTION('center_axis',(0.866025403784439,-0.5,0.));
#6186=DIRECTION('ref_axis',(0.5,0.866025403784439,0.));
#6187=DIRECTION('center_axis',(0.,0.,1.));
#6188=DIRECTION('ref_axis',(1.,0.,0.));
#6189=DIRECTION('center_axis',(0.,0.,1.));
#6190=DIRECTION('ref_axis',(1.,0.,0.));
#6191=DIRECTION('',(0.,0.,-1.));
#6192=DIRECTION('center_axis',(0.,0.,-1.));
#6193=DIRECTION('ref_axis',(1.,0.,0.));
#6194=DIRECTION('center_axis',(0.,0.,1.));
#6195=DIRECTION('ref_axis',(1.,0.,0.));
#6196=DIRECTION('',(0.,0.,-1.));
#6197=DIRECTION('center_axis',(0.,0.,1.));
#6198=DIRECTION('ref_axis',(1.,0.,0.));
#6199=DIRECTION('center_axis',(0.,0.,1.));
#6200=DIRECTION('ref_axis',(1.,0.,0.));
#7638=CARTESIAN_POINT('',(0.,0.,0.));
#7639=CARTESIAN_POINT('Origin',(0.35,0.8,8.5));
#7640=CARTESIAN_POINT('',(0.35,0.8,9.015));
#7641=CARTESIAN_POINT('Origin',(0.35,0.8,8.5));
#7642=CARTESIAN_POINT('',(1.,0.8,9.015));
#7643=CARTESIAN_POINT('',(0.35,0.8,9.015));
#7644=CARTESIAN_POINT('Origin',(1.,0.8,8.5));
#7645=CARTESIAN_POINT('Origin',(0.35,0.8,8.5));
#7646=CARTESIAN_POINT('',(0.35,0.606350832689629,8.9));
#7647=CARTESIAN_POINT('',(0.35,0.606350832689629,8.2));
#7648=CARTESIAN_POINT('',(0.35,0.606350832689629,8.2));
#7649=CARTESIAN_POINT('',(0.35,0.993649167310371,8.9));
#7650=CARTESIAN_POINT('',(0.35,0.8,8.9));
#7651=CARTESIAN_POINT('',(0.35,0.993649167310371,8.2));
#7652=CARTESIAN_POINT('',(0.35,0.993649167310371,8.2));
#7653=CARTESIAN_POINT('',(0.35,0.8,8.2));
#7654=CARTESIAN_POINT('Origin',(0.,0.8,8.9));
#7655=CARTESIAN_POINT('Origin',(0.,0.8,8.9));
#7656=CARTESIAN_POINT('',(-0.25,0.8,8.9));
#7657=CARTESIAN_POINT('Origin',(0.,0.8,8.9));
#7658=CARTESIAN_POINT('Origin',(0.,0.8,8.2));
#7659=CARTESIAN_POINT('Origin',(0.,0.8,8.2));
#7660=CARTESIAN_POINT('Origin',(0.,0.8,9.2));
#7661=CARTESIAN_POINT('',(-0.49,0.8,9.2));
#7662=CARTESIAN_POINT('Origin',(0.,0.8,9.2));
#7663=CARTESIAN_POINT('',(-0.49,0.8,9.4));
#7664=CARTESIAN_POINT('',(-0.49,0.8,9.2));
#7665=CARTESIAN_POINT('Origin',(0.,0.8,9.4));
#7666=CARTESIAN_POINT('Origin',(0.,0.8,9.4));
#7667=CARTESIAN_POINT('',(-0.25,0.8,9.4));
#7668=CARTESIAN_POINT('Origin',(0.,0.8,9.4));
#7669=CARTESIAN_POINT('Origin',(0.,0.8,9.2));
#7670=CARTESIAN_POINT('',(-0.25,0.8,9.2));
#7671=CARTESIAN_POINT('Origin',(0.,0.8,9.2));
#7672=CARTESIAN_POINT('Origin',(0.,0.8,8.8));
#7673=CARTESIAN_POINT('',(-0.25,0.8,8.8));
#7674=CARTESIAN_POINT('Origin',(0.,0.8,8.8));
#7675=CARTESIAN_POINT('',(-0.25,0.8,9.5));
#7676=CARTESIAN_POINT('',(-0.25,0.8,8.8));
#7677=CARTESIAN_POINT('Origin',(0.,0.8,9.5));
#7678=CARTESIAN_POINT('Origin',(0.,0.8,8.2));
#7679=CARTESIAN_POINT('',(-0.2,0.8,8.2));
#7680=CARTESIAN_POINT('Origin',(0.,0.8,8.2));
#7681=CARTESIAN_POINT('Origin',(0.,0.8,7.5));
#7682=CARTESIAN_POINT('',(-1.,0.782050807568877,7.5));
#7683=CARTESIAN_POINT('',(-0.505181485540923,-0.0749999999999997,7.5));
#7684=CARTESIAN_POINT('',(-1.01036297108185,0.8,7.5));
#7685=CARTESIAN_POINT('',(0.505181485540923,-0.075,7.5));
#7686=CARTESIAN_POINT('',(-0.505181485540923,-0.0749999999999997,7.5));
#7687=CARTESIAN_POINT('',(1.,0.782050807568877,7.5));
#7688=CARTESIAN_POINT('',(0.505181485540923,-0.075,7.5));
#7689=CARTESIAN_POINT('',(1.,-0.2,7.5));
#7690=CARTESIAN_POINT('',(1.,-0.2,7.5));
#7691=CARTESIAN_POINT('',(-1.,-0.2,7.5));
#7692=CARTESIAN_POINT('',(-1.,-0.2,7.5));
#7693=CARTESIAN_POINT('',(-1.,1.8,7.5));
#7694=CARTESIAN_POINT('Origin',(1.,1.8,7.5));
#7695=CARTESIAN_POINT('',(1.,1.8,7.5));
#7696=CARTESIAN_POINT('',(-1.,1.8,7.5));
#7697=CARTESIAN_POINT('',(1.,1.8,7.5));
#7698=CARTESIAN_POINT('',(-1.,1.8,9.5));
#7699=CARTESIAN_POINT('',(-1.,1.8,7.5));
#7700=CARTESIAN_POINT('',(1.,1.8,9.5));
#7701=CARTESIAN_POINT('',(1.,1.8,9.5));
#7702=CARTESIAN_POINT('',(1.,1.8,7.5));
#7703=CARTESIAN_POINT('Origin',(1.,-0.2,7.5));
#7704=CARTESIAN_POINT('',(1.,0.817949192431123,7.5));
#7705=CARTESIAN_POINT('',(1.,0.3,7.5));
#7706=CARTESIAN_POINT('',(1.,-0.2,7.5));
#7707=CARTESIAN_POINT('',(1.,-0.2,9.5));
#7708=CARTESIAN_POINT('',(1.,-0.2,9.5));
#7709=CARTESIAN_POINT('',(1.,-0.2,7.5));
#7710=CARTESIAN_POINT('Origin',(-1.,-0.2,7.5));
#7711=CARTESIAN_POINT('',(-1.,-0.2,9.5));
#7712=CARTESIAN_POINT('',(-1.,-0.2,9.5));
#7713=CARTESIAN_POINT('',(-1.,-0.2,7.5));
#7714=CARTESIAN_POINT('Origin',(-1.,1.8,7.5));
#7715=CARTESIAN_POINT('',(-1.,0.817949192431123,7.5));
#7716=CARTESIAN_POINT('',(-1.,1.8,7.5));
#7717=CARTESIAN_POINT('',(-1.,1.3,7.5));
#7718=CARTESIAN_POINT('',(-1.,1.8,9.5));
#7719=CARTESIAN_POINT('Origin',(0.,0.8,9.5));
#7720=CARTESIAN_POINT('Origin',(0.,0.8,7.5));
#7721=CARTESIAN_POINT('',(-0.505181485540922,1.675,7.5));
#7722=CARTESIAN_POINT('',(-0.505181485540922,1.675,7.5));
#7723=CARTESIAN_POINT('',(0.505181485540923,1.675,7.5));
#7724=CARTESIAN_POINT('',(1.01036297108185,0.8,7.5));
#7725=CARTESIAN_POINT('',(0.505181485540923,1.675,7.5));
#7726=CARTESIAN_POINT('Origin',(0.,0.8,7.5));
#7727=CARTESIAN_POINT('',(1.01036297108185,0.8,7.5));
#7728=CARTESIAN_POINT('',(0.505181485540923,-0.075,7.5));
#7729=CARTESIAN_POINT('',(1.01036297108185,0.8,7.5));
#7730=CARTESIAN_POINT('Origin',(0.,0.8,7.));
#7731=CARTESIAN_POINT('',(0.505181485540923,-0.075,7.));
#7732=CARTESIAN_POINT('',(1.01036297108185,0.8,7.));
#7733=CARTESIAN_POINT('',(0.505181485540923,-0.075,7.));
#7734=CARTESIAN_POINT('',(-0.505181485540923,-0.0749999999999997,7.));
#7735=CARTESIAN_POINT('',(-0.505181485540923,-0.0749999999999997,7.));
#7736=CARTESIAN_POINT('',(-1.01036297108185,0.8,7.));
#7737=CARTESIAN_POINT('',(-1.01036297108185,0.8,7.));
#7738=CARTESIAN_POINT('',(-0.505181485540922,1.675,7.));
#7739=CARTESIAN_POINT('',(-0.505181485540922,1.675,7.));
#7740=CARTESIAN_POINT('',(0.505181485540923,1.675,7.));
#7741=CARTESIAN_POINT('',(0.505181485540923,1.675,7.));
#7742=CARTESIAN_POINT('',(1.01036297108185,0.8,7.));
#7743=CARTESIAN_POINT('',(-0.685,0.8,7.));
#7744=CARTESIAN_POINT('Origin',(0.,0.8,7.));
#7745=CARTESIAN_POINT('Origin',(-0.505181485540923,-0.0749999999999997,
7.));
#7746=CARTESIAN_POINT('',(0.505181485540923,-0.075,7.));
#7747=CARTESIAN_POINT('',(-0.505181485540923,-0.0749999999999997,7.));
#7748=CARTESIAN_POINT('Origin',(-1.01036297108185,0.8,7.));
#7749=CARTESIAN_POINT('',(-1.01036297108185,0.8,7.5));
#7750=CARTESIAN_POINT('',(-1.01036297108185,0.8,7.5));
#7751=CARTESIAN_POINT('',(-1.01036297108185,0.8,7.));
#7752=CARTESIAN_POINT('Origin',(-0.505181485540922,1.675,7.));
#7753=CARTESIAN_POINT('',(-0.505181485540922,1.675,7.5));
#7754=CARTESIAN_POINT('',(-0.505181485540922,1.675,7.));
#7755=CARTESIAN_POINT('Origin',(0.505181485540923,1.675,7.));
#7756=CARTESIAN_POINT('',(0.505181485540923,1.675,7.));
#7757=CARTESIAN_POINT('Origin',(1.01036297108185,0.8,7.));
#7758=CARTESIAN_POINT('',(1.01036297108185,0.8,7.));
#7759=CARTESIAN_POINT('Origin',(0.505181485540923,-0.075,7.));
#7760=CARTESIAN_POINT('Origin',(0.,0.8,7.5));
#7761=CARTESIAN_POINT('Origin',(0.,0.8,5.8));
#7762=CARTESIAN_POINT('',(-0.2,0.8,5.8));
#7763=CARTESIAN_POINT('',(-0.2,0.8,5.8));
#7764=CARTESIAN_POINT('Origin',(0.,0.8,5.8));
#7765=CARTESIAN_POINT('Origin',(0.,0.8,5.8));
#7766=CARTESIAN_POINT('',(-0.685,0.8,5.8));
#7767=CARTESIAN_POINT('',(-0.685,0.8,5.8));
#7768=CARTESIAN_POINT('Origin',(0.,0.8,5.8));
#7769=CARTESIAN_POINT('Origin',(0.,0.8,5.8));
#9040=UNCERTAINTY_MEASURE_WITH_UNIT(LENGTH_MEASURE(0.001),#9103,
'DISTANCE_ACCURACY_VALUE',
'Maximum model space distance between geometric entities at asserted c
onnectivities');
#9069=UNCERTAINTY_MEASURE_WITH_UNIT(LENGTH_MEASURE(0.001),#9103,
'DISTANCE_ACCURACY_VALUE',
'Maximum model space distance between geometric entities at asserted c
onnectivities');
#9073=(
GEOMETRIC_REPRESENTATION_CONTEXT(3)
GLOBAL_UNCERTAINTY_ASSIGNED_CONTEXT((#9040))
GLOBAL_UNIT_ASSIGNED_CONTEXT((#9103,#9105,#9106))
REPRESENTATION_CONTEXT('','3D')
);
#9102=(
GEOMETRIC_REPRESENTATION_CONTEXT(3)
GLOBAL_UNCERTAINTY_ASSIGNED_CONTEXT((#9069))
GLOBAL_UNIT_ASSIGNED_CONTEXT((#9103,#9105,#9106))
REPRESENTATION_CONTEXT('','3D')
);
#9103=(
LENGTH_UNIT()
NAMED_UNIT(*)
SI_UNIT(.CENTI.,.METRE.)
);
#9105=(
NAMED_UNIT(*)
PLANE_ANGLE_UNIT()
SI_UNIT($,.RADIAN.)
);
#9106=(
NAMED_UNIT(*)
SI_UNIT($,.STERADIAN.)
SOLID_ANGLE_UNIT()
);
#9110=SHAPE_DEFINITION_REPRESENTATION(#9142,#9230);
#9142=PRODUCT_DEFINITION_SHAPE('',$,#9263);
#9230=SHAPE_REPRESENTATION('',(#5335),#9073);
#9259=PRODUCT_DEFINITION_CONTEXT('part definition',#9357,'design');
#9263=PRODUCT_DEFINITION('Needle flow-control fitting',
'Needle flow-control fitting',#9295,#9259);
#9295=PRODUCT_DEFINITION_FORMATION('',$,#9362);
#9357=APPLICATION_CONTEXT(
'Core Data for Automotive Mechanical Design Process');
#9358=PRODUCT_CONTEXT('part definition',#9357,'mechanical');
#9362=PRODUCT('Needle flow-control fitting',
'Needle flow-control fitting','Needle flow-control fitting',(#9358));
#9447=COLOUR_RGB('Sky Blue',0.24,0.69,0.87);
#9448=FILL_AREA_STYLE_COLOUR('',#9447);
#9449=FILL_AREA_STYLE('',(#9448));
#9450=SURFACE_STYLE_FILL_AREA(#9449);
#9451=SURFACE_SIDE_STYLE('',(#9450));
#9452=SURFACE_STYLE_USAGE(.BOTH.,#9451);
#9453=PRESENTATION_STYLE_ASSIGNMENT((#9452));
ENDSEC;
END-ISO-10303-21;
